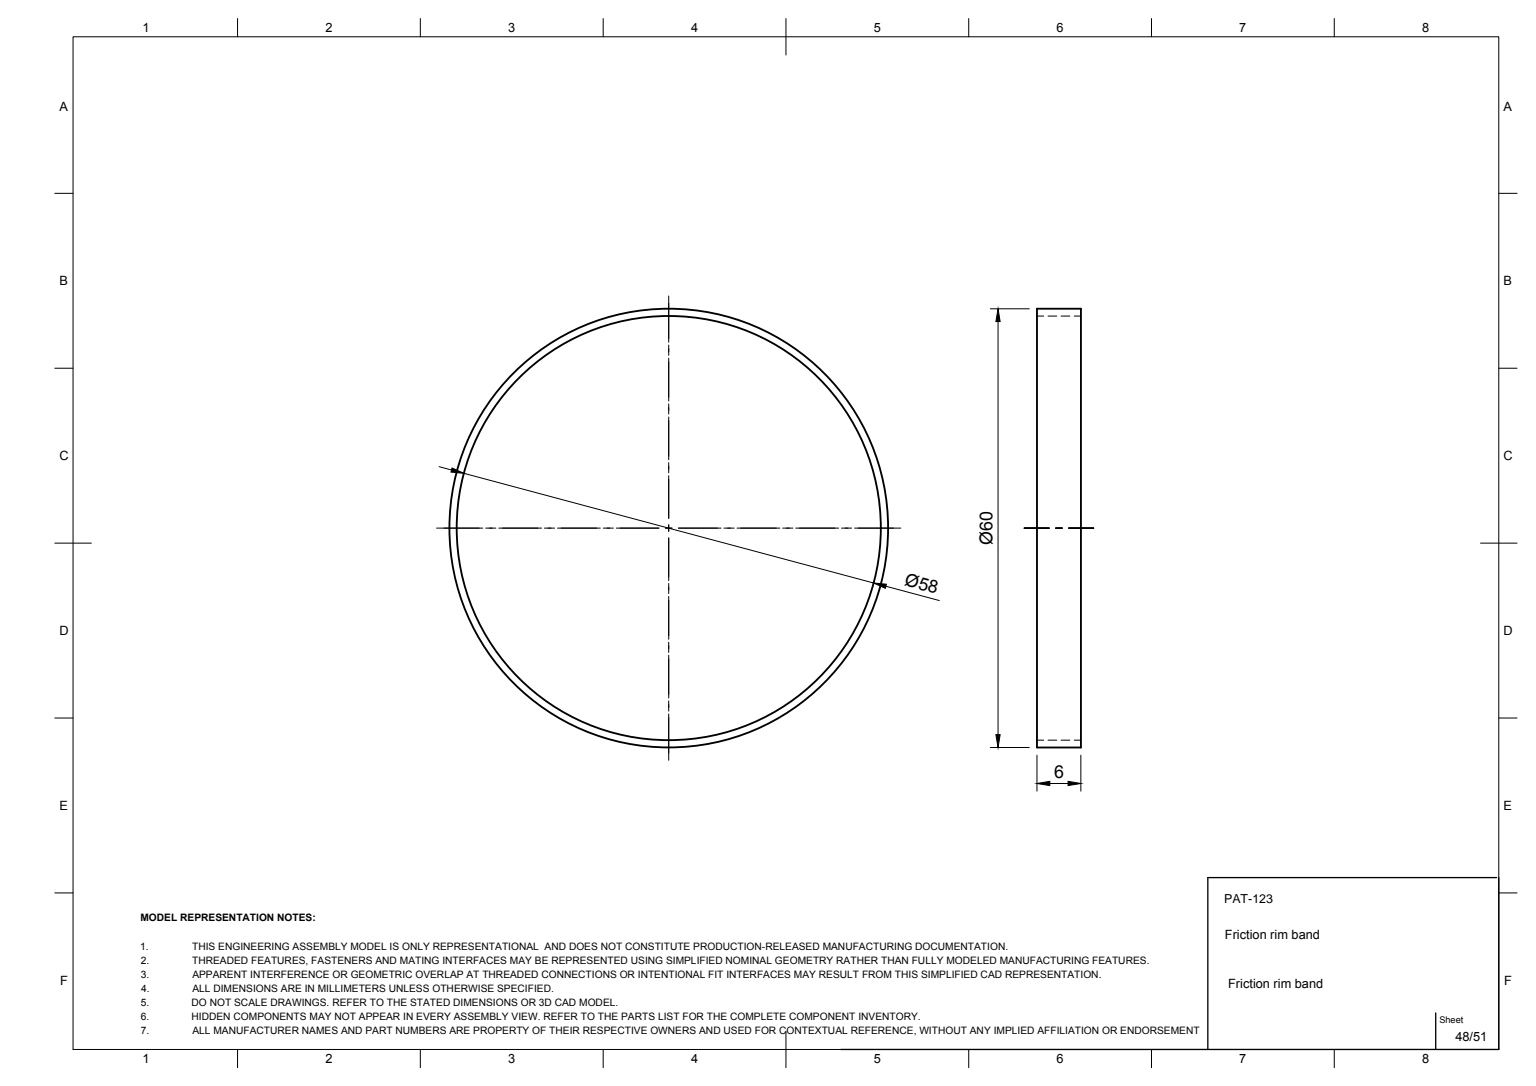
ISO-10303-21;
HEADER;
/* Generated by software containing ST-Developer
 * from STEP Tools, Inc. (www.steptools.com) 
 */

FILE_DESCRIPTION(
/* description */ ('Worm-less right-angle friction wheel drive'),
/* implementation_level */ '2;1');

FILE_NAME(
/* name */ 'Friction rim band.step',
/* time_stamp */ '2026-10-28T03:22:36-07:00',
/* author */ (''),
/* organization */ (''),
/* preprocessor_version */ 'ST-DEVELOPER v20.2',
/* originating_system */ 'Autodesk Translation Framework v15.17.0.0',
/* authorisation */ '');

FILE_SCHEMA (('AUTOMOTIVE_DESIGN { 1 0 10303 214 3 1 1 }'));
ENDSEC;

DATA;
#10=MECHANICAL_DESIGN_GEOMETRIC_PRESENTATION_REPRESENTATION('',(#659),#17046);
#558=SHAPE_REPRESENTATION_RELATIONSHIP('SRR','None',#17304,#605);
#605=ADVANCED_BREP_SHAPE_REPRESENTATION('',(#709),#17040);
#659=STYLED_ITEM('',(#17584),#709);
#709=MANIFOLD_SOLID_BREP('Body1',#8218);
#943=FACE_BOUND('',#2328,.T.);
#944=FACE_BOUND('',#2330,.T.);
#1177=PLANE('',#9687);
#1178=PLANE('',#9688);
#1631=FACE_OUTER_BOUND('',#2325,.T.);
#1632=FACE_OUTER_BOUND('',#2326,.T.);
#1633=FACE_OUTER_BOUND('',#2327,.T.);
#1634=FACE_OUTER_BOUND('',#2329,.T.);
#2325=EDGE_LOOP('',(#7332,#7333,#7334,#7335));
#2326=EDGE_LOOP('',(#7336,#7337,#7338,#7339));
#2327=EDGE_LOOP('',(#7340));
#2328=EDGE_LOOP('',(#7341));
#2329=EDGE_LOOP('',(#7342));
#2330=EDGE_LOOP('',(#7343));
#2855=LINE('',#16602,#3395);
#2856=LINE('',#16608,#3396);
#3395=VECTOR('',#12133,2.9);
#3396=VECTOR('',#12140,3.);
#3846=CIRCLE('',#9682,2.9);
#3847=CIRCLE('',#9683,2.9);
#3848=CIRCLE('',#9685,3.);
#3849=CIRCLE('',#9686,3.);
#4471=VERTEX_POINT('',#16599);
#4472=VERTEX_POINT('',#16601);
#4473=VERTEX_POINT('',#16605);
#4474=VERTEX_POINT('',#16607);
#5435=EDGE_CURVE('',#4471,#4471,#3846,.T.);
#5436=EDGE_CURVE('',#4471,#4472,#2855,.T.);
#5437=EDGE_CURVE('',#4472,#4472,#3847,.T.);
#5438=EDGE_CURVE('',#4473,#4473,#3848,.T.);
#5439=EDGE_CURVE('',#4473,#4474,#2856,.T.);
#5440=EDGE_CURVE('',#4474,#4474,#3849,.T.);
#7332=ORIENTED_EDGE('',*,*,#5435,.F.);
#7333=ORIENTED_EDGE('',*,*,#5436,.T.);
#7334=ORIENTED_EDGE('',*,*,#5437,.T.);
#7335=ORIENTED_EDGE('',*,*,#5436,.F.);
#7336=ORIENTED_EDGE('',*,*,#5438,.F.);
#7337=ORIENTED_EDGE('',*,*,#5439,.T.);
#7338=ORIENTED_EDGE('',*,*,#5440,.T.);
#7339=ORIENTED_EDGE('',*,*,#5439,.F.);
#7340=ORIENTED_EDGE('',*,*,#5438,.T.);
#7341=ORIENTED_EDGE('',*,*,#5435,.T.);
#7342=ORIENTED_EDGE('',*,*,#5440,.F.);
#7343=ORIENTED_EDGE('',*,*,#5437,.F.);
#7689=CYLINDRICAL_SURFACE('',#9681,2.9);
#7690=CYLINDRICAL_SURFACE('',#9684,3.);
#8123=ADVANCED_FACE('',(#1631),#7689,.F.);
#8124=ADVANCED_FACE('',(#1632),#7690,.T.);
#8125=ADVANCED_FACE('',(#1633,#943),#1177,.T.);
#8126=ADVANCED_FACE('',(#1634,#944),#1178,.F.);
#8218=CLOSED_SHELL('',(#8123,#8124,#8125,#8126));
#9680=AXIS2_PLACEMENT_3D('',#16597,#12127,#12128);
#9681=AXIS2_PLACEMENT_3D('',#16598,#12129,#12130);
#9682=AXIS2_PLACEMENT_3D('',#16600,#12131,#12132);
#9683=AXIS2_PLACEMENT_3D('',#16603,#12134,#12135);
#9684=AXIS2_PLACEMENT_3D('',#16604,#12136,#12137);
#9685=AXIS2_PLACEMENT_3D('',#16606,#12138,#12139);
#9686=AXIS2_PLACEMENT_3D('',#16609,#12141,#12142);
#9687=AXIS2_PLACEMENT_3D('',#16610,#12143,#12144);
#9688=AXIS2_PLACEMENT_3D('',#16611,#12145,#12146);
#12127=DIRECTION('axis',(0.,0.,1.));
#12128=DIRECTION('refdir',(1.,0.,0.));
#12129=DIRECTION('center_axis',(1.,0.,0.));
#12130=DIRECTION('ref_axis',(0.,0.,-1.));
#12131=DIRECTION('center_axis',(-1.,0.,0.));
#12132=DIRECTION('ref_axis',(0.,0.,-1.));
#12133=DIRECTION('',(-1.,0.,0.));
#12134=DIRECTION('center_axis',(-1.,0.,0.));
#12135=DIRECTION('ref_axis',(0.,0.,-1.));
#12136=DIRECTION('center_axis',(1.,0.,0.));
#12137=DIRECTION('ref_axis',(0.,0.,-1.));
#12138=DIRECTION('center_axis',(1.,0.,0.));
#12139=DIRECTION('ref_axis',(0.,0.,-1.));
#12140=DIRECTION('',(-1.,0.,0.));
#12141=DIRECTION('center_axis',(1.,0.,0.));
#12142=DIRECTION('ref_axis',(0.,0.,-1.));
#12143=DIRECTION('center_axis',(1.,0.,0.));
#12144=DIRECTION('ref_axis',(0.,0.,-1.));
#12145=DIRECTION('center_axis',(1.,0.,0.));
#12146=DIRECTION('ref_axis',(0.,0.,-1.));
#16597=CARTESIAN_POINT('',(0.,0.,0.));
#16598=CARTESIAN_POINT('Origin',(1.2,3.,7.));
#16599=CARTESIAN_POINT('',(1.8,3.,9.9));
#16600=CARTESIAN_POINT('Origin',(1.8,3.,7.));
#16601=CARTESIAN_POINT('',(1.2,3.,9.9));
#16602=CARTESIAN_POINT('',(1.2,3.,9.9));
#16603=CARTESIAN_POINT('Origin',(1.2,3.,7.));
#16604=CARTESIAN_POINT('Origin',(1.2,3.,7.));
#16605=CARTESIAN_POINT('',(1.8,3.,10.));
#16606=CARTESIAN_POINT('Origin',(1.8,3.,7.));
#16607=CARTESIAN_POINT('',(1.2,3.,10.));
#16608=CARTESIAN_POINT('',(1.2,3.,10.));
#16609=CARTESIAN_POINT('Origin',(1.2,3.,7.));
#16610=CARTESIAN_POINT('Origin',(1.8,3.,7.));
#16611=CARTESIAN_POINT('Origin',(1.2,3.,7.));
#16987=UNCERTAINTY_MEASURE_WITH_UNIT(LENGTH_MEASURE(0.001),#17047,
'DISTANCE_ACCURACY_VALUE',
'Maximum model space distance between geometric entities at asserted c
onnectivities');
#16993=UNCERTAINTY_MEASURE_WITH_UNIT(LENGTH_MEASURE(0.001),#17047,
'DISTANCE_ACCURACY_VALUE',
'Maximum model space distance between geometric entities at asserted c
onnectivities');
#17040=(
GEOMETRIC_REPRESENTATION_CONTEXT(3)
GLOBAL_UNCERTAINTY_ASSIGNED_CONTEXT((#16987))
GLOBAL_UNIT_ASSIGNED_CONTEXT((#17047,#17049,#17050))
REPRESENTATION_CONTEXT('','3D')
);
#17046=(
GEOMETRIC_REPRESENTATION_CONTEXT(3)
GLOBAL_UNCERTAINTY_ASSIGNED_CONTEXT((#16993))
GLOBAL_UNIT_ASSIGNED_CONTEXT((#17047,#17049,#17050))
REPRESENTATION_CONTEXT('','3D')
);
#17047=(
LENGTH_UNIT()
NAMED_UNIT(*)
SI_UNIT(.CENTI.,.METRE.)
);
#17049=(
NAMED_UNIT(*)
PLANE_ANGLE_UNIT()
SI_UNIT($,.RADIAN.)
);
#17050=(
NAMED_UNIT(*)
SI_UNIT($,.STERADIAN.)
SOLID_ANGLE_UNIT()
);
#17097=SHAPE_DEFINITION_REPRESENTATION(#17231,#17304);
#17231=PRODUCT_DEFINITION_SHAPE('',$,#17357);
#17304=SHAPE_REPRESENTATION('',(#9680),#17040);
#17310=PRODUCT_DEFINITION_CONTEXT('part definition',#17468,'design');
#17357=PRODUCT_DEFINITION('Friction rim band','Friction rim band',#17409,
#17310);
#17409=PRODUCT_DEFINITION_FORMATION('',$,#17516);
#17468=APPLICATION_CONTEXT(
'Core Data for Automotive Mechanical Design Process');
#17469=PRODUCT_CONTEXT('part definition',#17468,'mechanical');
#17516=PRODUCT('Friction rim band','Friction rim band',
'Friction rim band',(#17469));
#17578=COLOUR_RGB('Sky Blue',0.24,0.69,0.87);
#17579=FILL_AREA_STYLE_COLOUR('',#17578);
#17580=FILL_AREA_STYLE('',(#17579));
#17581=SURFACE_STYLE_FILL_AREA(#17580);
#17582=SURFACE_SIDE_STYLE('',(#17581));
#17583=SURFACE_STYLE_USAGE(.BOTH.,#17582);
#17584=PRESENTATION_STYLE_ASSIGNMENT((#17583));
ENDSEC;
END-ISO-10303-21;
